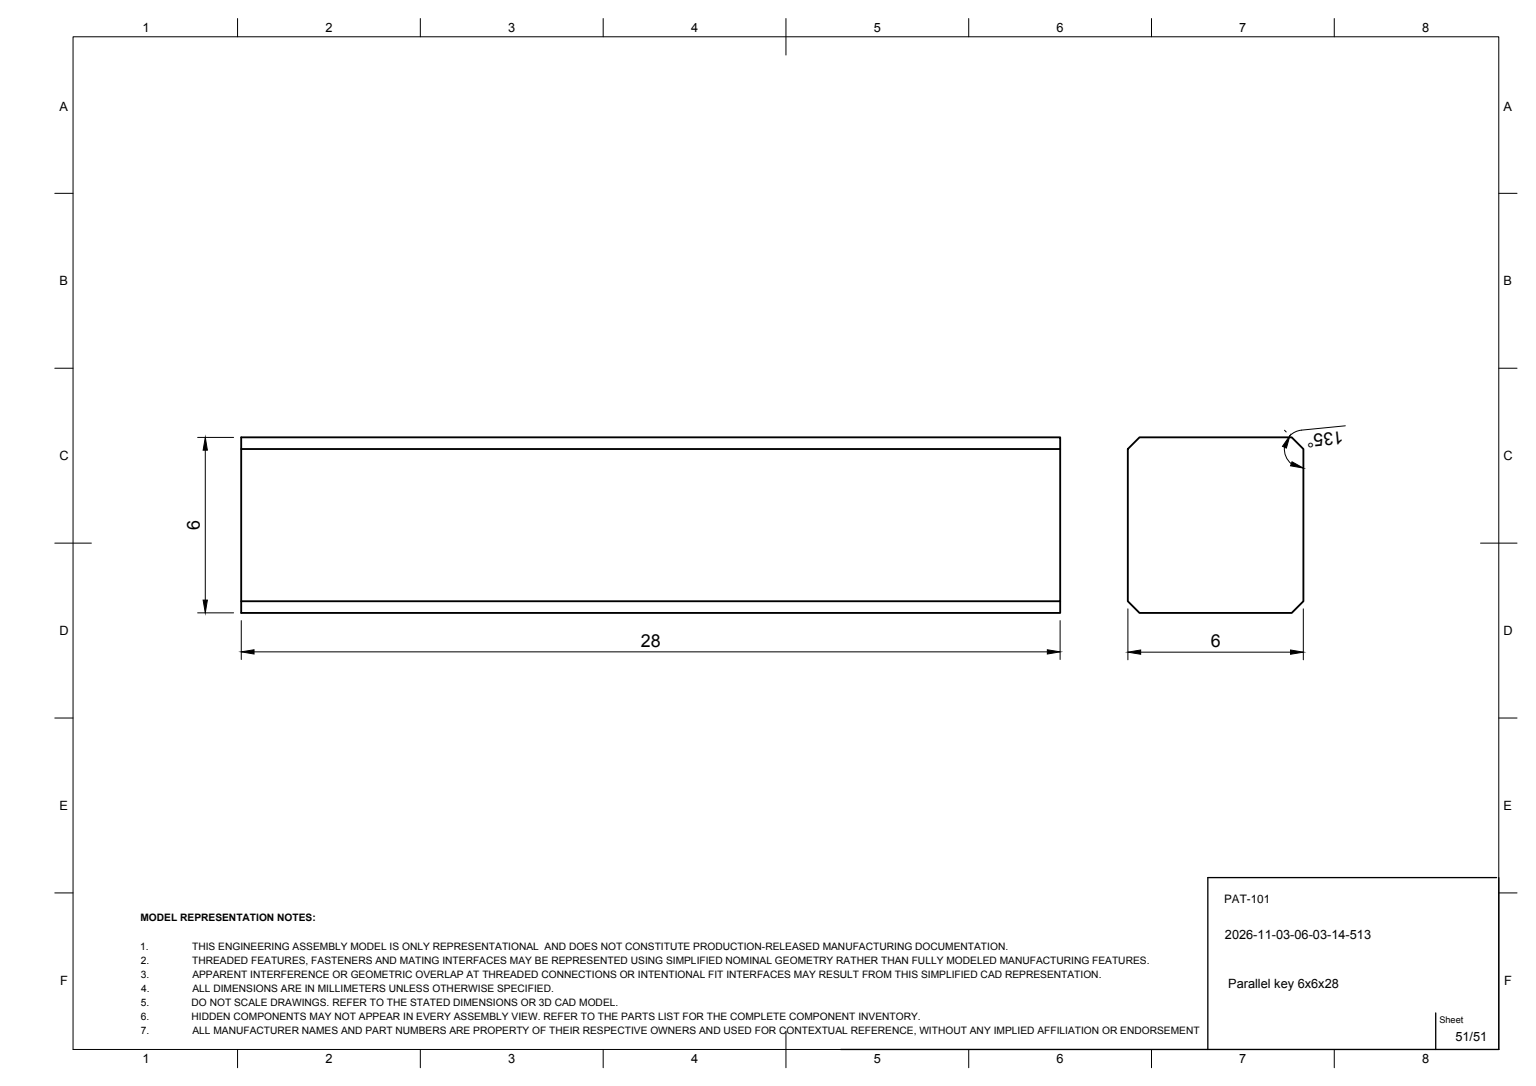
ISO-10303-21;
HEADER;
/* Generated by software containing ST-Developer
 * from STEP Tools, Inc. (www.steptools.com) 
 */

FILE_DESCRIPTION(
/* description */ ('Spur gear reduction stage 2-1 on bearing plates'),
/* implementation_level */ '2;1');

FILE_NAME(
/* name */ 'Parallel key 6x6x28.step',
/* time_stamp */ '2026-10-28T03:22:07-07:00',
/* author */ (''),
/* organization */ (''),
/* preprocessor_version */ 'ST-DEVELOPER v20.2',
/* originating_system */ 'Autodesk Translation Framework v15.17.0.0',
/* authorisation */ '');

FILE_SCHEMA (('AUTOMOTIVE_DESIGN { 1 0 10303 214 3 1 1 }'));
ENDSEC;

DATA;
#10=MECHANICAL_DESIGN_GEOMETRIC_PRESENTATION_REPRESENTATION('',(#1003),#53909);
#902=SHAPE_REPRESENTATION_RELATIONSHIP('SRR','None',#54133,#945);
#945=ADVANCED_BREP_SHAPE_REPRESENTATION('',(#1058),#53907);
#1003=STYLED_ITEM('',(#54397),#1058);
#1058=MANIFOLD_SOLID_BREP('Body1',#11330);
#1484=PLANE('',#12930);
#1485=PLANE('',#12931);
#1486=PLANE('',#12932);
#1487=PLANE('',#12933);
#1488=PLANE('',#12934);
#1489=PLANE('',#12935);
#1490=PLANE('',#12936);
#1491=PLANE('',#12937);
#1492=PLANE('',#12938);
#1493=PLANE('',#12939);
#2129=FACE_OUTER_BOUND('',#2954,.T.);
#2130=FACE_OUTER_BOUND('',#2955,.T.);
#2131=FACE_OUTER_BOUND('',#2956,.T.);
#2132=FACE_OUTER_BOUND('',#2957,.T.);
#2133=FACE_OUTER_BOUND('',#2958,.T.);
#2134=FACE_OUTER_BOUND('',#2959,.T.);
#2135=FACE_OUTER_BOUND('',#2960,.T.);
#2136=FACE_OUTER_BOUND('',#2961,.T.);
#2137=FACE_OUTER_BOUND('',#2962,.T.);
#2138=FACE_OUTER_BOUND('',#2963,.T.);
#2954=EDGE_LOOP('',(#10322,#10323,#10324,#10325,#10326,#10327,#10328,#10329));
#2955=EDGE_LOOP('',(#10330,#10331,#10332,#10333));
#2956=EDGE_LOOP('',(#10334,#10335,#10336,#10337));
#2957=EDGE_LOOP('',(#10338,#10339,#10340,#10341));
#2958=EDGE_LOOP('',(#10342,#10343,#10344,#10345));
#2959=EDGE_LOOP('',(#10346,#10347,#10348,#10349,#10350,#10351,#10352,#10353));
#2960=EDGE_LOOP('',(#10354,#10355,#10356,#10357));
#2961=EDGE_LOOP('',(#10358,#10359,#10360,#10361));
#2962=EDGE_LOOP('',(#10362,#10363,#10364,#10365));
#2963=EDGE_LOOP('',(#10366,#10367,#10368,#10369));
#3573=LINE('',#53684,#4214);
#3574=LINE('',#53686,#4215);
#3575=LINE('',#53688,#4216);
#3576=LINE('',#53690,#4217);
#3577=LINE('',#53692,#4218);
#3578=LINE('',#53694,#4219);
#3579=LINE('',#53696,#4220);
#3580=LINE('',#53697,#4221);
#3581=LINE('',#53700,#4222);
#3582=LINE('',#53702,#4223);
#3583=LINE('',#53703,#4224);
#3584=LINE('',#53706,#4225);
#3585=LINE('',#53707,#4226);
#3586=LINE('',#53710,#4227);
#3587=LINE('',#53711,#4228);
#3588=LINE('',#53714,#4229);
#3589=LINE('',#53715,#4230);
#3590=LINE('',#53719,#4231);
#3591=LINE('',#53720,#4232);
#3592=LINE('',#53722,#4233);
#3593=LINE('',#53723,#4234);
#3594=LINE('',#53725,#4235);
#3595=LINE('',#53727,#4236);
#3596=LINE('',#53729,#4237);
#4214=VECTOR('',#15828,1.);
#4215=VECTOR('',#15829,1.);
#4216=VECTOR('',#15830,1.);
#4217=VECTOR('',#15831,1.);
#4218=VECTOR('',#15832,1.);
#4219=VECTOR('',#15833,1.);
#4220=VECTOR('',#15834,1.);
#4221=VECTOR('',#15835,1.);
#4222=VECTOR('',#15838,1.);
#4223=VECTOR('',#15839,1.);
#4224=VECTOR('',#15840,1.);
#4225=VECTOR('',#15843,1.);
#4226=VECTOR('',#15844,1.);
#4227=VECTOR('',#15847,1.);
#4228=VECTOR('',#15848,1.);
#4229=VECTOR('',#15851,1.);
#4230=VECTOR('',#15852,1.);
#4231=VECTOR('',#15855,1.);
#4232=VECTOR('',#15856,1.);
#4233=VECTOR('',#15857,1.);
#4234=VECTOR('',#15858,1.);
#4235=VECTOR('',#15861,1.);
#4236=VECTOR('',#15864,1.);
#4237=VECTOR('',#15867,1.);
#5786=VERTEX_POINT('',#53682);
#5787=VERTEX_POINT('',#53683);
#5788=VERTEX_POINT('',#53685);
#5789=VERTEX_POINT('',#53687);
#5790=VERTEX_POINT('',#53689);
#5791=VERTEX_POINT('',#53691);
#5792=VERTEX_POINT('',#53693);
#5793=VERTEX_POINT('',#53695);
#5794=VERTEX_POINT('',#53699);
#5795=VERTEX_POINT('',#53701);
#5796=VERTEX_POINT('',#53705);
#5797=VERTEX_POINT('',#53709);
#5798=VERTEX_POINT('',#53713);
#5799=VERTEX_POINT('',#53717);
#5800=VERTEX_POINT('',#53718);
#5801=VERTEX_POINT('',#53721);
#7303=EDGE_CURVE('',#5786,#5787,#3573,.T.);
#7304=EDGE_CURVE('',#5788,#5786,#3574,.T.);
#7305=EDGE_CURVE('',#5789,#5788,#3575,.T.);
#7306=EDGE_CURVE('',#5790,#5789,#3576,.T.);
#7307=EDGE_CURVE('',#5791,#5790,#3577,.T.);
#7308=EDGE_CURVE('',#5792,#5791,#3578,.T.);
#7309=EDGE_CURVE('',#5793,#5792,#3579,.T.);
#7310=EDGE_CURVE('',#5787,#5793,#3580,.T.);
#7311=EDGE_CURVE('',#5790,#5794,#3581,.T.);
#7312=EDGE_CURVE('',#5794,#5795,#3582,.T.);
#7313=EDGE_CURVE('',#5795,#5791,#3583,.T.);
#7314=EDGE_CURVE('',#5796,#5789,#3584,.T.);
#7315=EDGE_CURVE('',#5796,#5794,#3585,.T.);
#7316=EDGE_CURVE('',#5788,#5797,#3586,.T.);
#7317=EDGE_CURVE('',#5797,#5796,#3587,.T.);
#7318=EDGE_CURVE('',#5798,#5786,#3588,.T.);
#7319=EDGE_CURVE('',#5798,#5797,#3589,.T.);
#7320=EDGE_CURVE('',#5799,#5800,#3590,.T.);
#7321=EDGE_CURVE('',#5795,#5799,#3591,.T.);
#7322=EDGE_CURVE('',#5801,#5798,#3592,.T.);
#7323=EDGE_CURVE('',#5800,#5801,#3593,.T.);
#7324=EDGE_CURVE('',#5792,#5799,#3594,.T.);
#7325=EDGE_CURVE('',#5787,#5801,#3595,.T.);
#7326=EDGE_CURVE('',#5800,#5793,#3596,.T.);
#10322=ORIENTED_EDGE('',*,*,#7303,.F.);
#10323=ORIENTED_EDGE('',*,*,#7304,.F.);
#10324=ORIENTED_EDGE('',*,*,#7305,.F.);
#10325=ORIENTED_EDGE('',*,*,#7306,.F.);
#10326=ORIENTED_EDGE('',*,*,#7307,.F.);
#10327=ORIENTED_EDGE('',*,*,#7308,.F.);
#10328=ORIENTED_EDGE('',*,*,#7309,.F.);
#10329=ORIENTED_EDGE('',*,*,#7310,.F.);
#10330=ORIENTED_EDGE('',*,*,#7307,.T.);
#10331=ORIENTED_EDGE('',*,*,#7311,.T.);
#10332=ORIENTED_EDGE('',*,*,#7312,.T.);
#10333=ORIENTED_EDGE('',*,*,#7313,.T.);
#10334=ORIENTED_EDGE('',*,*,#7306,.T.);
#10335=ORIENTED_EDGE('',*,*,#7314,.F.);
#10336=ORIENTED_EDGE('',*,*,#7315,.T.);
#10337=ORIENTED_EDGE('',*,*,#7311,.F.);
#10338=ORIENTED_EDGE('',*,*,#7305,.T.);
#10339=ORIENTED_EDGE('',*,*,#7316,.T.);
#10340=ORIENTED_EDGE('',*,*,#7317,.T.);
#10341=ORIENTED_EDGE('',*,*,#7314,.T.);
#10342=ORIENTED_EDGE('',*,*,#7304,.T.);
#10343=ORIENTED_EDGE('',*,*,#7318,.F.);
#10344=ORIENTED_EDGE('',*,*,#7319,.T.);
#10345=ORIENTED_EDGE('',*,*,#7316,.F.);
#10346=ORIENTED_EDGE('',*,*,#7320,.F.);
#10347=ORIENTED_EDGE('',*,*,#7321,.F.);
#10348=ORIENTED_EDGE('',*,*,#7312,.F.);
#10349=ORIENTED_EDGE('',*,*,#7315,.F.);
#10350=ORIENTED_EDGE('',*,*,#7317,.F.);
#10351=ORIENTED_EDGE('',*,*,#7319,.F.);
#10352=ORIENTED_EDGE('',*,*,#7322,.F.);
#10353=ORIENTED_EDGE('',*,*,#7323,.F.);
#10354=ORIENTED_EDGE('',*,*,#7308,.T.);
#10355=ORIENTED_EDGE('',*,*,#7313,.F.);
#10356=ORIENTED_EDGE('',*,*,#7321,.T.);
#10357=ORIENTED_EDGE('',*,*,#7324,.F.);
#10358=ORIENTED_EDGE('',*,*,#7303,.T.);
#10359=ORIENTED_EDGE('',*,*,#7325,.T.);
#10360=ORIENTED_EDGE('',*,*,#7322,.T.);
#10361=ORIENTED_EDGE('',*,*,#7318,.T.);
#10362=ORIENTED_EDGE('',*,*,#7309,.T.);
#10363=ORIENTED_EDGE('',*,*,#7324,.T.);
#10364=ORIENTED_EDGE('',*,*,#7320,.T.);
#10365=ORIENTED_EDGE('',*,*,#7326,.T.);
#10366=ORIENTED_EDGE('',*,*,#7310,.T.);
#10367=ORIENTED_EDGE('',*,*,#7326,.F.);
#10368=ORIENTED_EDGE('',*,*,#7323,.T.);
#10369=ORIENTED_EDGE('',*,*,#7325,.F.);
#11249=ADVANCED_FACE('',(#2129),#1484,.F.);
#11250=ADVANCED_FACE('',(#2130),#1485,.T.);
#11251=ADVANCED_FACE('',(#2131),#1486,.T.);
#11252=ADVANCED_FACE('',(#2132),#1487,.T.);
#11253=ADVANCED_FACE('',(#2133),#1488,.T.);
#11254=ADVANCED_FACE('',(#2134),#1489,.T.);
#11255=ADVANCED_FACE('',(#2135),#1490,.F.);
#11256=ADVANCED_FACE('',(#2136),#1491,.T.);
#11257=ADVANCED_FACE('',(#2137),#1492,.T.);
#11258=ADVANCED_FACE('',(#2138),#1493,.T.);
#11330=CLOSED_SHELL('',(#11249,#11250,#11251,#11252,#11253,#11254,#11255,
#11256,#11257,#11258));
#12929=AXIS2_PLACEMENT_3D('',#53680,#15824,#15825);
#12930=AXIS2_PLACEMENT_3D('',#53681,#15826,#15827);
#12931=AXIS2_PLACEMENT_3D('',#53698,#15836,#15837);
#12932=AXIS2_PLACEMENT_3D('',#53704,#15841,#15842);
#12933=AXIS2_PLACEMENT_3D('',#53708,#15845,#15846);
#12934=AXIS2_PLACEMENT_3D('',#53712,#15849,#15850);
#12935=AXIS2_PLACEMENT_3D('',#53716,#15853,#15854);
#12936=AXIS2_PLACEMENT_3D('',#53724,#15859,#15860);
#12937=AXIS2_PLACEMENT_3D('',#53726,#15862,#15863);
#12938=AXIS2_PLACEMENT_3D('',#53728,#15865,#15866);
#12939=AXIS2_PLACEMENT_3D('',#53730,#15868,#15869);
#15824=DIRECTION('axis',(0.,0.,1.));
#15825=DIRECTION('refdir',(1.,0.,0.));
#15826=DIRECTION('center_axis',(1.,0.,0.));
#15827=DIRECTION('ref_axis',(0.,0.,-1.));
#15828=DIRECTION('',(0.,-0.707106781186547,-0.707106781186548));
#15829=DIRECTION('',(0.,-1.,0.));
#15830=DIRECTION('',(0.,-0.707106781186547,0.707106781186548));
#15831=DIRECTION('',(0.,0.,1.));
#15832=DIRECTION('',(0.,0.707106781186547,0.707106781186548));
#15833=DIRECTION('',(0.,1.,0.));
#15834=DIRECTION('',(0.,0.707106781186547,-0.707106781186548));
#15835=DIRECTION('',(0.,0.,-1.));
#15836=DIRECTION('center_axis',(0.,0.707106781186548,-0.707106781186547));
#15837=DIRECTION('ref_axis',(-1.,0.,0.));
#15838=DIRECTION('',(1.,0.,0.));
#15839=DIRECTION('',(0.,-0.707106781186547,-0.707106781186548));
#15840=DIRECTION('',(-1.,0.,0.));
#15841=DIRECTION('center_axis',(0.,1.,0.));
#15842=DIRECTION('ref_axis',(-1.,0.,0.));
#15843=DIRECTION('',(-1.,0.,0.));
#15844=DIRECTION('',(0.,0.,-1.));
#15845=DIRECTION('center_axis',(0.,0.707106781186548,0.707106781186547));
#15846=DIRECTION('ref_axis',(1.,0.,0.));
#15847=DIRECTION('',(1.,0.,0.));
#15848=DIRECTION('',(0.,0.707106781186547,-0.707106781186548));
#15849=DIRECTION('center_axis',(0.,0.,1.));
#15850=DIRECTION('ref_axis',(1.,0.,0.));
#15851=DIRECTION('',(-1.,0.,0.));
#15852=DIRECTION('',(0.,1.,0.));
#15853=DIRECTION('center_axis',(1.,0.,0.));
#15854=DIRECTION('ref_axis',(0.,0.,-1.));
#15855=DIRECTION('',(0.,-0.707106781186547,0.707106781186548));
#15856=DIRECTION('',(0.,-1.,0.));
#15857=DIRECTION('',(0.,0.707106781186547,0.707106781186548));
#15858=DIRECTION('',(0.,0.,1.));
#15859=DIRECTION('center_axis',(0.,0.,1.));
#15860=DIRECTION('ref_axis',(1.,0.,0.));
#15861=DIRECTION('',(1.,0.,0.));
#15862=DIRECTION('center_axis',(0.,-0.707106781186548,0.707106781186547));
#15863=DIRECTION('ref_axis',(1.,0.,0.));
#15864=DIRECTION('',(1.,0.,0.));
#15865=DIRECTION('center_axis',(0.,-0.707106781186548,-0.707106781186547));
#15866=DIRECTION('ref_axis',(-1.,0.,0.));
#15867=DIRECTION('',(-1.,0.,0.));
#15868=DIRECTION('center_axis',(0.,-1.,0.));
#15869=DIRECTION('ref_axis',(1.,0.,0.));
#53680=CARTESIAN_POINT('',(0.,0.,0.));
#53681=CARTESIAN_POINT('Origin',(-1.4,0.,0.35));
#53682=CARTESIAN_POINT('',(-1.4,-0.26,0.6));
#53683=CARTESIAN_POINT('',(-1.4,-0.3,0.56));
#53684=CARTESIAN_POINT('',(-1.4,-0.2675,0.5925));
#53685=CARTESIAN_POINT('',(-1.4,0.26,0.6));
#53686=CARTESIAN_POINT('',(-1.4,0.,0.6));
#53687=CARTESIAN_POINT('',(-1.4,0.3,0.56));
#53688=CARTESIAN_POINT('',(-1.4,0.2675,0.5925));
#53689=CARTESIAN_POINT('',(-1.4,0.3,0.04));
#53690=CARTESIAN_POINT('',(-1.4,0.3,0.175));
#53691=CARTESIAN_POINT('',(-1.4,0.26,0.));
#53692=CARTESIAN_POINT('',(-1.4,0.2925,0.0325));
#53693=CARTESIAN_POINT('',(-1.4,-0.26,0.));
#53694=CARTESIAN_POINT('',(-1.4,0.,0.));
#53695=CARTESIAN_POINT('',(-1.4,-0.3,0.04));
#53696=CARTESIAN_POINT('',(-1.4,-0.2925,0.0325));
#53697=CARTESIAN_POINT('',(-1.4,-0.3,0.175));
#53698=CARTESIAN_POINT('Origin',(0.75,0.28,0.02));
#53699=CARTESIAN_POINT('',(1.4,0.3,0.04));
#53700=CARTESIAN_POINT('',(0.75,0.3,0.04));
#53701=CARTESIAN_POINT('',(1.4,0.26,0.));
#53702=CARTESIAN_POINT('',(1.4,0.2925,0.0325));
#53703=CARTESIAN_POINT('',(0.75,0.26,0.));
#53704=CARTESIAN_POINT('Origin',(1.5,0.3,0.));
#53705=CARTESIAN_POINT('',(1.4,0.3,0.56));
#53706=CARTESIAN_POINT('',(0.75,0.3,0.56));
#53707=CARTESIAN_POINT('',(1.4,0.3,0.175));
#53708=CARTESIAN_POINT('Origin',(0.75,0.28,0.58));
#53709=CARTESIAN_POINT('',(1.4,0.26,0.6));
#53710=CARTESIAN_POINT('',(0.75,0.26,0.6));
#53711=CARTESIAN_POINT('',(1.4,0.2675,0.5925));
#53712=CARTESIAN_POINT('Origin',(0.,0.,0.6));
#53713=CARTESIAN_POINT('',(1.4,-0.26,0.6));
#53714=CARTESIAN_POINT('',(-0.75,-0.26,0.6));
#53715=CARTESIAN_POINT('',(1.4,0.,0.6));
#53716=CARTESIAN_POINT('Origin',(1.4,0.,0.35));
#53717=CARTESIAN_POINT('',(1.4,-0.26,0.));
#53718=CARTESIAN_POINT('',(1.4,-0.3,0.04));
#53719=CARTESIAN_POINT('',(1.4,-0.2925,0.0325));
#53720=CARTESIAN_POINT('',(1.4,0.,0.));
#53721=CARTESIAN_POINT('',(1.4,-0.3,0.56));
#53722=CARTESIAN_POINT('',(1.4,-0.2675,0.5925));
#53723=CARTESIAN_POINT('',(1.4,-0.3,0.175));
#53724=CARTESIAN_POINT('Origin',(0.,0.,0.));
#53725=CARTESIAN_POINT('',(-0.75,-0.26,0.));
#53726=CARTESIAN_POINT('Origin',(-0.75,-0.28,0.58));
#53727=CARTESIAN_POINT('',(-0.75,-0.3,0.56));
#53728=CARTESIAN_POINT('Origin',(-0.75,-0.28,0.02));
#53729=CARTESIAN_POINT('',(-0.75,-0.3,0.04));
#53730=CARTESIAN_POINT('Origin',(-1.5,-0.3,0.));
#53857=UNCERTAINTY_MEASURE_WITH_UNIT(LENGTH_MEASURE(0.001),#53910,
'DISTANCE_ACCURACY_VALUE',
'Maximum model space distance between geometric entities at asserted c
onnectivities');
#53859=UNCERTAINTY_MEASURE_WITH_UNIT(LENGTH_MEASURE(0.001),#53910,
'DISTANCE_ACCURACY_VALUE',
'Maximum model space distance between geometric entities at asserted c
onnectivities');
#53907=(
GEOMETRIC_REPRESENTATION_CONTEXT(3)
GLOBAL_UNCERTAINTY_ASSIGNED_CONTEXT((#53857))
GLOBAL_UNIT_ASSIGNED_CONTEXT((#53910,#53912,#53913))
REPRESENTATION_CONTEXT('','3D')
);
#53909=(
GEOMETRIC_REPRESENTATION_CONTEXT(3)
GLOBAL_UNCERTAINTY_ASSIGNED_CONTEXT((#53859))
GLOBAL_UNIT_ASSIGNED_CONTEXT((#53910,#53912,#53913))
REPRESENTATION_CONTEXT('','3D')
);
#53910=(
LENGTH_UNIT()
NAMED_UNIT(*)
SI_UNIT(.CENTI.,.METRE.)
);
#53912=(
NAMED_UNIT(*)
PLANE_ANGLE_UNIT()
SI_UNIT($,.RADIAN.)
);
#53913=(
NAMED_UNIT(*)
SI_UNIT($,.STERADIAN.)
SOLID_ANGLE_UNIT()
);
#53961=SHAPE_DEFINITION_REPRESENTATION(#54059,#54133);
#54059=PRODUCT_DEFINITION_SHAPE('',$,#54183);
#54133=SHAPE_REPRESENTATION('',(#12929),#53907);
#54135=PRODUCT_DEFINITION_CONTEXT('part definition',#54284,'design');
#54183=PRODUCT_DEFINITION('Parallel key 6x6x28','Parallel key 6x6x28',#54232,
#54135);
#54232=PRODUCT_DEFINITION_FORMATION('',$,#54333);
#54284=APPLICATION_CONTEXT(
'Core Data for Automotive Mechanical Design Process');
#54285=PRODUCT_CONTEXT('part definition',#54284,'mechanical');
#54333=PRODUCT('Parallel key 6x6x28','Parallel key 6x6x28',
'Parallel key 6x6x28',(#54285));
#54391=COLOUR_RGB('Grey',0.48,0.52,0.57);
#54392=FILL_AREA_STYLE_COLOUR('',#54391);
#54393=FILL_AREA_STYLE('',(#54392));
#54394=SURFACE_STYLE_FILL_AREA(#54393);
#54395=SURFACE_SIDE_STYLE('',(#54394));
#54396=SURFACE_STYLE_USAGE(.BOTH.,#54395);
#54397=PRESENTATION_STYLE_ASSIGNMENT((#54396));
ENDSEC;
END-ISO-10303-21;
